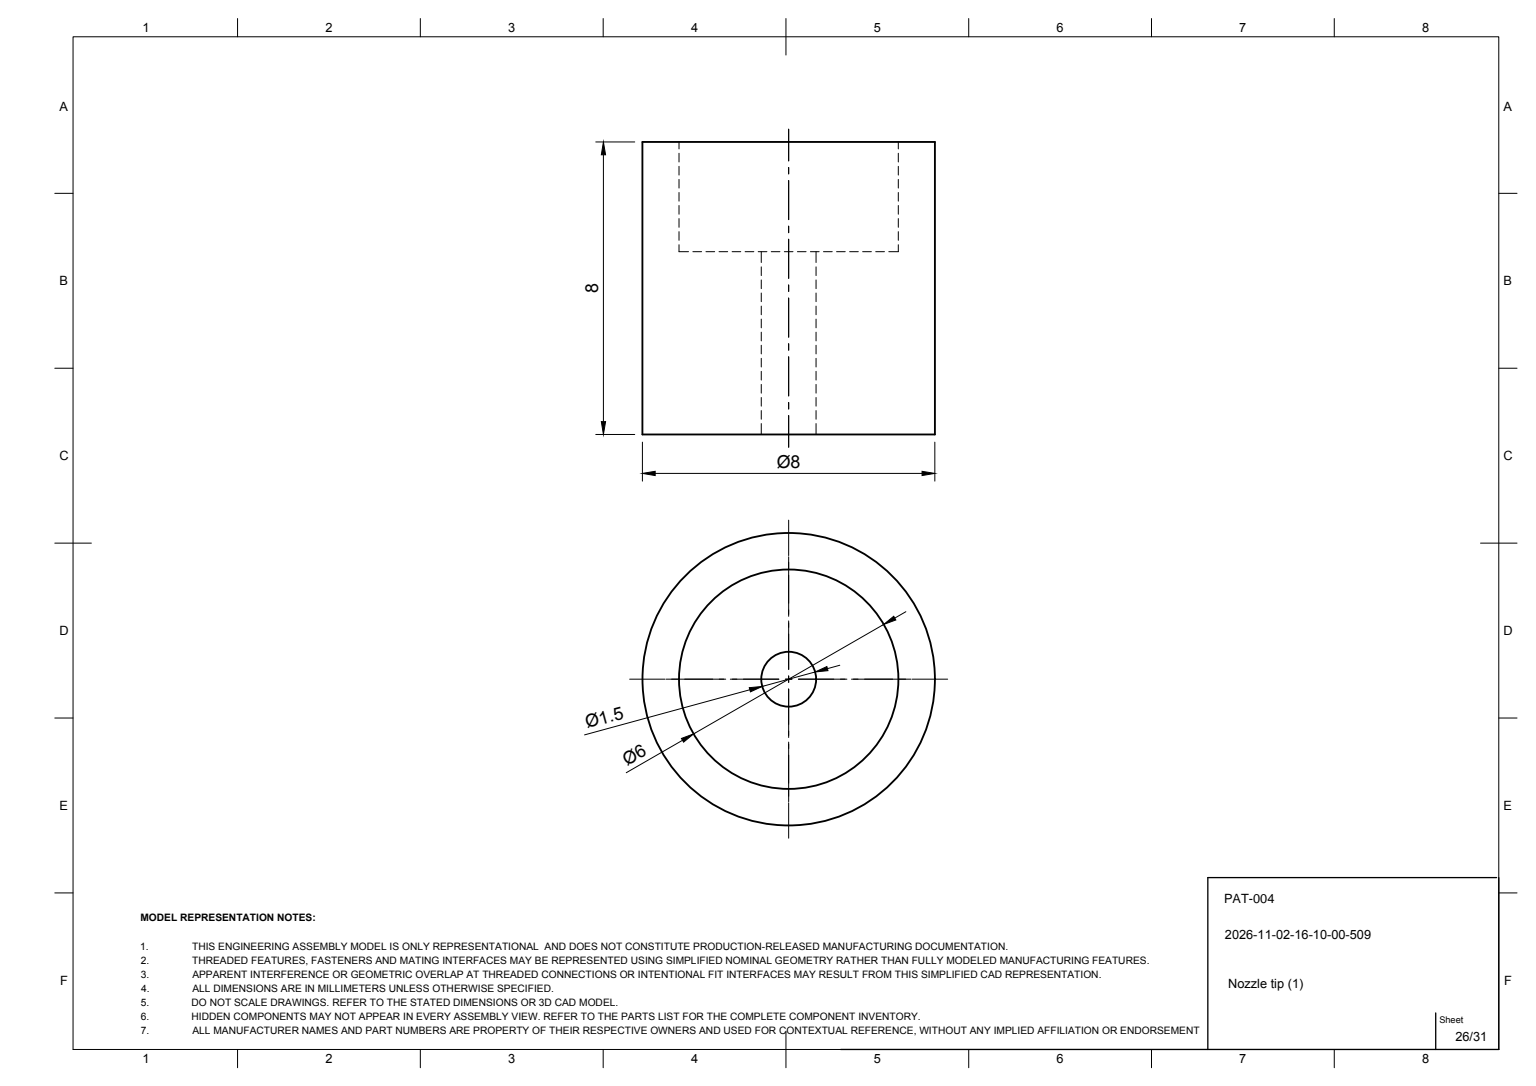
ISO-10303-21;
HEADER;
/* Generated by software containing ST-Developer
 * from STEP Tools, Inc. (www.steptools.com) 
 */

FILE_DESCRIPTION(
/* description */ ('Air blow-off nozzle station'),
/* implementation_level */ '2;1');

FILE_NAME(
/* name */ 'Nozzle tip (1).step',
/* time_stamp */ '2026-10-27T10:53:54-07:00',
/* author */ (''),
/* organization */ (''),
/* preprocessor_version */ 'ST-DEVELOPER v20.2',
/* originating_system */ 'Autodesk Translation Framework v15.17.0.0',
/* authorisation */ '');

FILE_SCHEMA (('AUTOMOTIVE_DESIGN { 1 0 10303 214 3 1 1 }'));
ENDSEC;

DATA;
#10=MECHANICAL_DESIGN_GEOMETRIC_PRESENTATION_REPRESENTATION('',(#256),#7897);
#206=SHAPE_REPRESENTATION_RELATIONSHIP('SRR','None',#8022,#231);
#231=ADVANCED_BREP_SHAPE_REPRESENTATION('',(#279),#7889);
#256=STYLED_ITEM('',(#8213),#279);
#279=MANIFOLD_SOLID_BREP('Body1',#4307);
#350=FACE_BOUND('',#1074,.T.);
#351=FACE_BOUND('',#1078,.T.);
#352=FACE_BOUND('',#1080,.T.);
#515=PLANE('',#4966);
#516=PLANE('',#4973);
#517=PLANE('',#4974);
#751=FACE_OUTER_BOUND('',#1072,.T.);
#752=FACE_OUTER_BOUND('',#1073,.T.);
#753=FACE_OUTER_BOUND('',#1075,.T.);
#754=FACE_OUTER_BOUND('',#1076,.T.);
#755=FACE_OUTER_BOUND('',#1077,.T.);
#756=FACE_OUTER_BOUND('',#1079,.T.);
#1072=EDGE_LOOP('',(#3807,#3808,#3809,#3810));
#1073=EDGE_LOOP('',(#3811));
#1074=EDGE_LOOP('',(#3812));
#1075=EDGE_LOOP('',(#3813,#3814,#3815,#3816));
#1076=EDGE_LOOP('',(#3817,#3818,#3819,#3820));
#1077=EDGE_LOOP('',(#3821));
#1078=EDGE_LOOP('',(#3822));
#1079=EDGE_LOOP('',(#3823));
#1080=EDGE_LOOP('',(#3824));
#1455=LINE('',#7640,#1809);
#1456=LINE('',#7647,#1810);
#1457=LINE('',#7653,#1811);
#1809=VECTOR('',#6141,0.3);
#1810=VECTOR('',#6150,0.075);
#1811=VECTOR('',#6157,0.4);
#1968=CIRCLE('',#4964,0.3);
#1969=CIRCLE('',#4965,0.3);
#1970=CIRCLE('',#4967,0.075);
#1971=CIRCLE('',#4969,0.075);
#1972=CIRCLE('',#4971,0.4);
#1973=CIRCLE('',#4972,0.4);
#2314=VERTEX_POINT('',#7637);
#2315=VERTEX_POINT('',#7639);
#2316=VERTEX_POINT('',#7643);
#2317=VERTEX_POINT('',#7646);
#2318=VERTEX_POINT('',#7650);
#2319=VERTEX_POINT('',#7652);
#2821=EDGE_CURVE('',#2314,#2314,#1968,.T.);
#2822=EDGE_CURVE('',#2314,#2315,#1455,.T.);
#2823=EDGE_CURVE('',#2315,#2315,#1969,.T.);
#2824=EDGE_CURVE('',#2316,#2316,#1970,.T.);
#2825=EDGE_CURVE('',#2316,#2317,#1456,.T.);
#2826=EDGE_CURVE('',#2317,#2317,#1971,.T.);
#2827=EDGE_CURVE('',#2318,#2318,#1972,.T.);
#2828=EDGE_CURVE('',#2318,#2319,#1457,.T.);
#2829=EDGE_CURVE('',#2319,#2319,#1973,.T.);
#3807=ORIENTED_EDGE('',*,*,#2821,.F.);
#3808=ORIENTED_EDGE('',*,*,#2822,.T.);
#3809=ORIENTED_EDGE('',*,*,#2823,.F.);
#3810=ORIENTED_EDGE('',*,*,#2822,.F.);
#3811=ORIENTED_EDGE('',*,*,#2821,.T.);
#3812=ORIENTED_EDGE('',*,*,#2824,.F.);
#3813=ORIENTED_EDGE('',*,*,#2824,.T.);
#3814=ORIENTED_EDGE('',*,*,#2825,.T.);
#3815=ORIENTED_EDGE('',*,*,#2826,.T.);
#3816=ORIENTED_EDGE('',*,*,#2825,.F.);
#3817=ORIENTED_EDGE('',*,*,#2827,.F.);
#3818=ORIENTED_EDGE('',*,*,#2828,.T.);
#3819=ORIENTED_EDGE('',*,*,#2829,.T.);
#3820=ORIENTED_EDGE('',*,*,#2828,.F.);
#3821=ORIENTED_EDGE('',*,*,#2827,.T.);
#3822=ORIENTED_EDGE('',*,*,#2823,.T.);
#3823=ORIENTED_EDGE('',*,*,#2829,.F.);
#3824=ORIENTED_EDGE('',*,*,#2826,.F.);
#4011=CYLINDRICAL_SURFACE('',#4963,0.3);
#4012=CYLINDRICAL_SURFACE('',#4968,0.075);
#4013=CYLINDRICAL_SURFACE('',#4970,0.4);
#4241=ADVANCED_FACE('',(#751),#4011,.F.);
#4242=ADVANCED_FACE('',(#752,#350),#515,.T.);
#4243=ADVANCED_FACE('',(#753),#4012,.F.);
#4244=ADVANCED_FACE('',(#754),#4013,.T.);
#4245=ADVANCED_FACE('',(#755,#351),#516,.T.);
#4246=ADVANCED_FACE('',(#756,#352),#517,.F.);
#4307=CLOSED_SHELL('',(#4241,#4242,#4243,#4244,#4245,#4246));
#4962=AXIS2_PLACEMENT_3D('',#7635,#6135,#6136);
#4963=AXIS2_PLACEMENT_3D('',#7636,#6137,#6138);
#4964=AXIS2_PLACEMENT_3D('',#7638,#6139,#6140);
#4965=AXIS2_PLACEMENT_3D('',#7641,#6142,#6143);
#4966=AXIS2_PLACEMENT_3D('',#7642,#6144,#6145);
#4967=AXIS2_PLACEMENT_3D('',#7644,#6146,#6147);
#4968=AXIS2_PLACEMENT_3D('',#7645,#6148,#6149);
#4969=AXIS2_PLACEMENT_3D('',#7648,#6151,#6152);
#4970=AXIS2_PLACEMENT_3D('',#7649,#6153,#6154);
#4971=AXIS2_PLACEMENT_3D('',#7651,#6155,#6156);
#4972=AXIS2_PLACEMENT_3D('',#7654,#6158,#6159);
#4973=AXIS2_PLACEMENT_3D('',#7655,#6160,#6161);
#4974=AXIS2_PLACEMENT_3D('',#7656,#6162,#6163);
#6135=DIRECTION('axis',(0.,0.,1.));
#6136=DIRECTION('refdir',(1.,0.,0.));
#6137=DIRECTION('center_axis',(0.,1.,0.));
#6138=DIRECTION('ref_axis',(1.,0.,0.));
#6139=DIRECTION('center_axis',(0.,1.,0.));
#6140=DIRECTION('ref_axis',(1.,0.,0.));
#6141=DIRECTION('',(0.,1.,0.));
#6142=DIRECTION('center_axis',(0.,-1.,0.));
#6143=DIRECTION('ref_axis',(1.,0.,0.));
#6144=DIRECTION('center_axis',(0.,1.,0.));
#6145=DIRECTION('ref_axis',(1.,0.,0.));
#6146=DIRECTION('center_axis',(0.,1.,0.));
#6147=DIRECTION('ref_axis',(1.,0.,0.));
#6148=DIRECTION('center_axis',(0.,1.,0.));
#6149=DIRECTION('ref_axis',(1.,0.,0.));
#6150=DIRECTION('',(0.,-1.,0.));
#6151=DIRECTION('center_axis',(0.,-1.,0.));
#6152=DIRECTION('ref_axis',(1.,0.,0.));
#6153=DIRECTION('center_axis',(0.,1.,0.));
#6154=DIRECTION('ref_axis',(1.,0.,0.));
#6155=DIRECTION('center_axis',(0.,1.,0.));
#6156=DIRECTION('ref_axis',(1.,0.,0.));
#6157=DIRECTION('',(0.,-1.,0.));
#6158=DIRECTION('center_axis',(0.,1.,0.));
#6159=DIRECTION('ref_axis',(1.,0.,0.));
#6160=DIRECTION('center_axis',(0.,1.,0.));
#6161=DIRECTION('ref_axis',(1.,0.,0.));
#6162=DIRECTION('center_axis',(0.,1.,0.));
#6163=DIRECTION('ref_axis',(1.,0.,0.));
#7635=CARTESIAN_POINT('',(0.,0.,0.));
#7636=CARTESIAN_POINT('Origin',(0.,-7.2,23.));
#7637=CARTESIAN_POINT('',(-0.3,-7.2,23.));
#7638=CARTESIAN_POINT('Origin',(0.,-7.2,23.));
#7639=CARTESIAN_POINT('',(-0.3,-6.9,23.));
#7640=CARTESIAN_POINT('',(-0.3,-7.2,23.));
#7641=CARTESIAN_POINT('Origin',(0.,-6.9,23.));
#7642=CARTESIAN_POINT('Origin',(0.,-7.2,23.));
#7643=CARTESIAN_POINT('',(-0.075,-7.2,23.));
#7644=CARTESIAN_POINT('Origin',(0.,-7.2,23.));
#7645=CARTESIAN_POINT('Origin',(0.,-7.7,23.));
#7646=CARTESIAN_POINT('',(-0.075,-7.7,23.));
#7647=CARTESIAN_POINT('',(-0.075,-7.7,23.));
#7648=CARTESIAN_POINT('Origin',(0.,-7.7,23.));
#7649=CARTESIAN_POINT('Origin',(0.,-7.7,23.));
#7650=CARTESIAN_POINT('',(-0.4,-6.9,23.));
#7651=CARTESIAN_POINT('Origin',(0.,-6.9,23.));
#7652=CARTESIAN_POINT('',(-0.4,-7.7,23.));
#7653=CARTESIAN_POINT('',(-0.4,-7.7,23.));
#7654=CARTESIAN_POINT('Origin',(0.,-7.7,23.));
#7655=CARTESIAN_POINT('Origin',(0.,-6.9,23.));
#7656=CARTESIAN_POINT('Origin',(0.,-7.7,23.));
#7857=UNCERTAINTY_MEASURE_WITH_UNIT(LENGTH_MEASURE(0.001),#7898,
'DISTANCE_ACCURACY_VALUE',
'Maximum model space distance between geometric entities at asserted c
onnectivities');
#7865=UNCERTAINTY_MEASURE_WITH_UNIT(LENGTH_MEASURE(0.001),#7898,
'DISTANCE_ACCURACY_VALUE',
'Maximum model space distance between geometric entities at asserted c
onnectivities');
#7889=(
GEOMETRIC_REPRESENTATION_CONTEXT(3)
GLOBAL_UNCERTAINTY_ASSIGNED_CONTEXT((#7857))
GLOBAL_UNIT_ASSIGNED_CONTEXT((#7898,#7900,#7901))
REPRESENTATION_CONTEXT('','3D')
);
#7897=(
GEOMETRIC_REPRESENTATION_CONTEXT(3)
GLOBAL_UNCERTAINTY_ASSIGNED_CONTEXT((#7865))
GLOBAL_UNIT_ASSIGNED_CONTEXT((#7898,#7900,#7901))
REPRESENTATION_CONTEXT('','3D')
);
#7898=(
LENGTH_UNIT()
NAMED_UNIT(*)
SI_UNIT(.CENTI.,.METRE.)
);
#7900=(
NAMED_UNIT(*)
PLANE_ANGLE_UNIT()
SI_UNIT($,.RADIAN.)
);
#7901=(
NAMED_UNIT(*)
SI_UNIT($,.STERADIAN.)
SOLID_ANGLE_UNIT()
);
#7925=SHAPE_DEFINITION_REPRESENTATION(#7973,#8022);
#7973=PRODUCT_DEFINITION_SHAPE('',$,#8054);
#8022=SHAPE_REPRESENTATION('',(#4962),#7889);
#8030=PRODUCT_DEFINITION_CONTEXT('part definition',#8125,'design');
#8054=PRODUCT_DEFINITION('Nozzle tip (1)','Nozzle tip (1)',#8085,#8030);
#8085=PRODUCT_DEFINITION_FORMATION('',$,#8150);
#8125=APPLICATION_CONTEXT(
'Core Data for Automotive Mechanical Design Process');
#8126=PRODUCT_CONTEXT('part definition',#8125,'mechanical');
#8150=PRODUCT('Nozzle tip (1)','Nozzle tip (1)','Nozzle tip (1)',(#8126));
#8207=COLOUR_RGB('Sky Blue',0.24,0.69,0.87);
#8208=FILL_AREA_STYLE_COLOUR('',#8207);
#8209=FILL_AREA_STYLE('',(#8208));
#8210=SURFACE_STYLE_FILL_AREA(#8209);
#8211=SURFACE_SIDE_STYLE('',(#8210));
#8212=SURFACE_STYLE_USAGE(.BOTH.,#8211);
#8213=PRESENTATION_STYLE_ASSIGNMENT((#8212));
ENDSEC;
END-ISO-10303-21;
